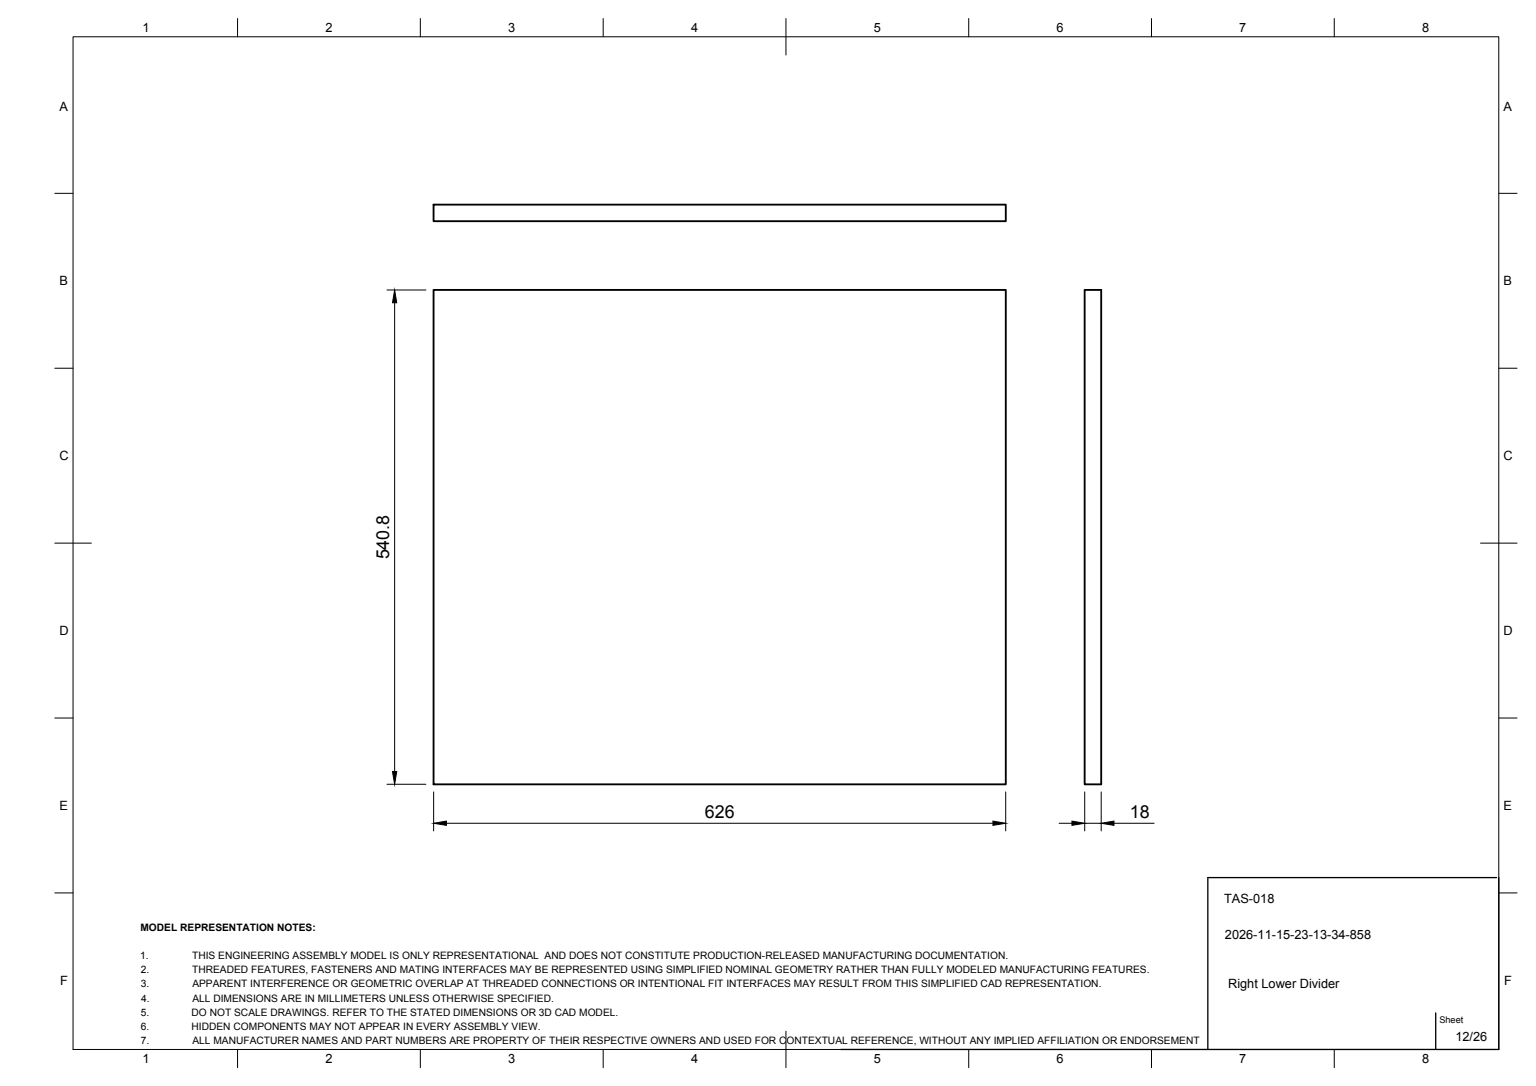
ISO-10303-21;
HEADER;
/* Generated by software containing ST-Developer
 * from STEP Tools, Inc. (www.steptools.com) 
 */

FILE_DESCRIPTION(
/* description */ (''),
/* implementation_level */ '2;1');

FILE_NAME(
/* name */ 'Right Lower Divider.step',
/* time_stamp */ '2026-11-15T15:17:57-08:00',
/* author */ (''),
/* organization */ (''),
/* preprocessor_version */ 'ST-DEVELOPER v20.2',
/* originating_system */ 'Autodesk Translation Framework v15.17.0.0',
/* authorisation */ '');

FILE_SCHEMA (('AUTOMOTIVE_DESIGN { 1 0 10303 214 3 1 1 }'));
ENDSEC;

DATA;
#10=MECHANICAL_DESIGN_GEOMETRIC_PRESENTATION_REPRESENTATION('',(#187),#3723);
#139=SHAPE_REPRESENTATION_RELATIONSHIP('SRR','None',#3820,#163);
#163=ADVANCED_BREP_SHAPE_REPRESENTATION('',(#211),#3709);
#187=STYLED_ITEM('',(#3946),#211);
#211=MANIFOLD_SOLID_BREP('Body1',#2035);
#282=FACE_OUTER_BOUND('',#408,.T.);
#283=FACE_OUTER_BOUND('',#409,.T.);
#284=FACE_OUTER_BOUND('',#410,.T.);
#285=FACE_OUTER_BOUND('',#411,.T.);
#286=FACE_OUTER_BOUND('',#412,.T.);
#287=FACE_OUTER_BOUND('',#413,.T.);
#408=EDGE_LOOP('',(#1533,#1534,#1535,#1536));
#409=EDGE_LOOP('',(#1537,#1538,#1539,#1540));
#410=EDGE_LOOP('',(#1541,#1542,#1543,#1544));
#411=EDGE_LOOP('',(#1545,#1546,#1547,#1548));
#412=EDGE_LOOP('',(#1549,#1550,#1551,#1552));
#413=EDGE_LOOP('',(#1553,#1554,#1555,#1556));
#586=LINE('',#3362,#808);
#587=LINE('',#3364,#809);
#588=LINE('',#3366,#810);
#589=LINE('',#3367,#811);
#590=LINE('',#3371,#812);
#591=LINE('',#3372,#813);
#592=LINE('',#3373,#814);
#593=LINE('',#3376,#815);
#594=LINE('',#3378,#816);
#595=LINE('',#3379,#817);
#596=LINE('',#3381,#818);
#597=LINE('',#3382,#819);
#808=VECTOR('',#2760,21.2913385826772);
#809=VECTOR('',#2761,24.6456692913386);
#810=VECTOR('',#2762,21.2913385826772);
#811=VECTOR('',#2763,24.6456692913386);
#812=VECTOR('',#2766,21.2913385826772);
#813=VECTOR('',#2767,0.708661417322836);
#814=VECTOR('',#2768,0.708661417322836);
#815=VECTOR('',#2771,24.6456692913386);
#816=VECTOR('',#2772,24.6456692913386);
#817=VECTOR('',#2773,21.2913385826772);
#818=VECTOR('',#2776,0.708661417322836);
#819=VECTOR('',#2777,0.708661417322836);
#995=VERTEX_POINT('',#3360);
#996=VERTEX_POINT('',#3361);
#997=VERTEX_POINT('',#3363);
#998=VERTEX_POINT('',#3365);
#999=VERTEX_POINT('',#3369);
#1000=VERTEX_POINT('',#3370);
#1001=VERTEX_POINT('',#3375);
#1002=VERTEX_POINT('',#3377);
#1188=EDGE_CURVE('',#995,#996,#586,.T.);
#1189=EDGE_CURVE('',#995,#997,#587,.T.);
#1190=EDGE_CURVE('',#997,#998,#588,.T.);
#1191=EDGE_CURVE('',#996,#998,#589,.T.);
#1192=EDGE_CURVE('',#999,#1000,#590,.T.);
#1193=EDGE_CURVE('',#999,#995,#591,.T.);
#1194=EDGE_CURVE('',#1000,#996,#592,.T.);
#1195=EDGE_CURVE('',#999,#1001,#593,.T.);
#1196=EDGE_CURVE('',#1000,#1002,#594,.T.);
#1197=EDGE_CURVE('',#1001,#1002,#595,.T.);
#1198=EDGE_CURVE('',#1001,#997,#596,.T.);
#1199=EDGE_CURVE('',#1002,#998,#597,.T.);
#1533=ORIENTED_EDGE('',*,*,#1188,.F.);
#1534=ORIENTED_EDGE('',*,*,#1189,.T.);
#1535=ORIENTED_EDGE('',*,*,#1190,.T.);
#1536=ORIENTED_EDGE('',*,*,#1191,.F.);
#1537=ORIENTED_EDGE('',*,*,#1192,.F.);
#1538=ORIENTED_EDGE('',*,*,#1193,.T.);
#1539=ORIENTED_EDGE('',*,*,#1188,.T.);
#1540=ORIENTED_EDGE('',*,*,#1194,.F.);
#1541=ORIENTED_EDGE('',*,*,#1195,.F.);
#1542=ORIENTED_EDGE('',*,*,#1192,.T.);
#1543=ORIENTED_EDGE('',*,*,#1196,.T.);
#1544=ORIENTED_EDGE('',*,*,#1197,.F.);
#1545=ORIENTED_EDGE('',*,*,#1198,.F.);
#1546=ORIENTED_EDGE('',*,*,#1197,.T.);
#1547=ORIENTED_EDGE('',*,*,#1199,.T.);
#1548=ORIENTED_EDGE('',*,*,#1190,.F.);
#1549=ORIENTED_EDGE('',*,*,#1191,.T.);
#1550=ORIENTED_EDGE('',*,*,#1199,.F.);
#1551=ORIENTED_EDGE('',*,*,#1196,.F.);
#1552=ORIENTED_EDGE('',*,*,#1194,.T.);
#1553=ORIENTED_EDGE('',*,*,#1189,.F.);
#1554=ORIENTED_EDGE('',*,*,#1193,.F.);
#1555=ORIENTED_EDGE('',*,*,#1195,.T.);
#1556=ORIENTED_EDGE('',*,*,#1198,.T.);
#1835=PLANE('',#2387);
#1836=PLANE('',#2388);
#1837=PLANE('',#2389);
#1838=PLANE('',#2390);
#1839=PLANE('',#2391);
#1840=PLANE('',#2392);
#1956=ADVANCED_FACE('',(#282),#1835,.T.);
#1957=ADVANCED_FACE('',(#283),#1836,.T.);
#1958=ADVANCED_FACE('',(#284),#1837,.F.);
#1959=ADVANCED_FACE('',(#285),#1838,.F.);
#1960=ADVANCED_FACE('',(#286),#1839,.F.);
#1961=ADVANCED_FACE('',(#287),#1840,.T.);
#2035=CLOSED_SHELL('',(#1956,#1957,#1958,#1959,#1960,#1961));
#2386=AXIS2_PLACEMENT_3D('',#3358,#2756,#2757);
#2387=AXIS2_PLACEMENT_3D('',#3359,#2758,#2759);
#2388=AXIS2_PLACEMENT_3D('',#3368,#2764,#2765);
#2389=AXIS2_PLACEMENT_3D('',#3374,#2769,#2770);
#2390=AXIS2_PLACEMENT_3D('',#3380,#2774,#2775);
#2391=AXIS2_PLACEMENT_3D('',#3383,#2778,#2779);
#2392=AXIS2_PLACEMENT_3D('',#3384,#2780,#2781);
#2756=DIRECTION('axis',(0.,0.,1.));
#2757=DIRECTION('refdir',(1.,0.,0.));
#2758=DIRECTION('center_axis',(-1.,0.,0.));
#2759=DIRECTION('ref_axis',(0.,0.,1.));
#2760=DIRECTION('',(0.,0.,-1.));
#2761=DIRECTION('',(0.,1.,0.));
#2762=DIRECTION('',(0.,0.,-1.));
#2763=DIRECTION('',(0.,1.,0.));
#2764=DIRECTION('center_axis',(0.,-1.,0.));
#2765=DIRECTION('ref_axis',(0.,0.,-1.));
#2766=DIRECTION('',(0.,0.,-1.));
#2767=DIRECTION('',(-1.,0.,0.));
#2768=DIRECTION('',(-1.,0.,0.));
#2769=DIRECTION('center_axis',(-1.,0.,0.));
#2770=DIRECTION('ref_axis',(0.,0.,1.));
#2771=DIRECTION('',(0.,1.,0.));
#2772=DIRECTION('',(0.,1.,0.));
#2773=DIRECTION('',(0.,0.,-1.));
#2774=DIRECTION('center_axis',(0.,-1.,0.));
#2775=DIRECTION('ref_axis',(0.,0.,-1.));
#2776=DIRECTION('',(-1.,0.,0.));
#2777=DIRECTION('',(-1.,0.,0.));
#2778=DIRECTION('center_axis',(0.,0.,1.));
#2779=DIRECTION('ref_axis',(1.,0.,0.));
#2780=DIRECTION('center_axis',(0.,0.,1.));
#2781=DIRECTION('ref_axis',(1.,0.,0.));
#3358=CARTESIAN_POINT('',(0.,0.,0.));
#3359=CARTESIAN_POINT('Origin',(22.9370078740157,0.,46.6558556092144));
#3360=CARTESIAN_POINT('',(22.9370078740157,4.64566929133858,22.));
#3361=CARTESIAN_POINT('',(22.9370078740157,4.64566929133858,0.708661417322834));
#3362=CARTESIAN_POINT('',(22.9370078740157,4.64566929133858,22.));
#3363=CARTESIAN_POINT('',(22.9370078740157,29.2913385826772,22.));
#3364=CARTESIAN_POINT('',(22.9370078740157,4.64566929133858,22.));
#3365=CARTESIAN_POINT('',(22.9370078740157,29.2913385826772,0.708661417322834));
#3366=CARTESIAN_POINT('',(22.9370078740157,29.2913385826772,22.));
#3367=CARTESIAN_POINT('',(22.9370078740157,4.64566929133858,0.708661417322834));
#3368=CARTESIAN_POINT('Origin',(0.,4.64566929133858,46.6558556092144));
#3369=CARTESIAN_POINT('',(23.6456692913386,4.64566929133858,22.));
#3370=CARTESIAN_POINT('',(23.6456692913386,4.64566929133858,0.708661417322834));
#3371=CARTESIAN_POINT('',(23.6456692913386,4.64566929133858,22.));
#3372=CARTESIAN_POINT('',(23.6456692913386,4.64566929133858,22.));
#3373=CARTESIAN_POINT('',(23.6456692913386,4.64566929133858,0.708661417322834));
#3374=CARTESIAN_POINT('Origin',(23.6456692913386,0.,46.6558556092144));
#3375=CARTESIAN_POINT('',(23.6456692913386,29.2913385826772,22.));
#3376=CARTESIAN_POINT('',(23.6456692913386,4.64566929133858,22.));
#3377=CARTESIAN_POINT('',(23.6456692913386,29.2913385826772,0.708661417322834));
#3378=CARTESIAN_POINT('',(23.6456692913386,4.64566929133858,0.708661417322834));
#3379=CARTESIAN_POINT('',(23.6456692913386,29.2913385826772,22.));
#3380=CARTESIAN_POINT('Origin',(0.,29.2913385826772,46.6558556092144));
#3381=CARTESIAN_POINT('',(23.6456692913386,29.2913385826772,22.));
#3382=CARTESIAN_POINT('',(23.6456692913386,29.2913385826772,0.708661417322834));
#3383=CARTESIAN_POINT('Origin',(0.,0.,0.708661417322834));
#3384=CARTESIAN_POINT('Origin',(0.,0.,22.));
#3682=UNCERTAINTY_MEASURE_WITH_UNIT(LENGTH_MEASURE(0.000393700787401575),
#3725,'DISTANCE_ACCURACY_VALUE',
'Maximum model space distance between geometric entities at asserted c
onnectivities');
#3696=UNCERTAINTY_MEASURE_WITH_UNIT(LENGTH_MEASURE(0.000393700787401575),
#3725,'DISTANCE_ACCURACY_VALUE',
'Maximum model space distance between geometric entities at asserted c
onnectivities');
#3709=(
GEOMETRIC_REPRESENTATION_CONTEXT(3)
GLOBAL_UNCERTAINTY_ASSIGNED_CONTEXT((#3682))
GLOBAL_UNIT_ASSIGNED_CONTEXT((#3725,#3729,#3730))
REPRESENTATION_CONTEXT('','3D')
);
#3723=(
GEOMETRIC_REPRESENTATION_CONTEXT(3)
GLOBAL_UNCERTAINTY_ASSIGNED_CONTEXT((#3696))
GLOBAL_UNIT_ASSIGNED_CONTEXT((#3725,#3729,#3730))
REPRESENTATION_CONTEXT('','3D')
);
#3724=DIMENSIONAL_EXPONENTS(1.,0.,0.,0.,0.,0.,0.);
#3725=(
CONVERSION_BASED_UNIT('inch',#3728)
LENGTH_UNIT()
NAMED_UNIT(#3724)
);
#3726=(
LENGTH_UNIT()
NAMED_UNIT(*)
SI_UNIT(.MILLI.,.METRE.)
);
#3728=LENGTH_MEASURE_WITH_UNIT(LENGTH_MEASURE(25.4),#3726);
#3729=(
NAMED_UNIT(*)
PLANE_ANGLE_UNIT()
SI_UNIT($,.RADIAN.)
);
#3730=(
NAMED_UNIT(*)
SI_UNIT($,.STERADIAN.)
SOLID_ANGLE_UNIT()
);
#3743=SHAPE_DEFINITION_REPRESENTATION(#3770,#3820);
#3770=PRODUCT_DEFINITION_SHAPE('',$,#3847);
#3820=SHAPE_REPRESENTATION('',(#2386),#3709);
#3834=PRODUCT_DEFINITION_CONTEXT('part definition',#3914,'design');
#3847=PRODUCT_DEFINITION('2026-11-15-23-13-34-858',
'Right Lower Divider',#3873,#3834);
#3873=PRODUCT_DEFINITION_FORMATION('',$,#3928);
#3914=APPLICATION_CONTEXT(
'Core Data for Automotive Mechanical Design Process');
#3915=PRODUCT_CONTEXT('part definition',#3914,'mechanical');
#3928=PRODUCT('2026-11-15-23-13-34-858','Right Lower Divider',$,(#3915));
#3946=PRESENTATION_STYLE_ASSIGNMENT((#3954));
#3954=SURFACE_STYLE_USAGE(.BOTH.,#3962);
#3962=SURFACE_SIDE_STYLE('',(#3970));
#3970=SURFACE_STYLE_FILL_AREA(#3978);
#3978=FILL_AREA_STYLE('Gray',(#3986));
#3986=FILL_AREA_STYLE_COLOUR('Gray',#3994);
#3994=COLOUR_RGB('Gray',0.501960784313725,0.501960784313725,0.501960784313725);
ENDSEC;
END-ISO-10303-21;
